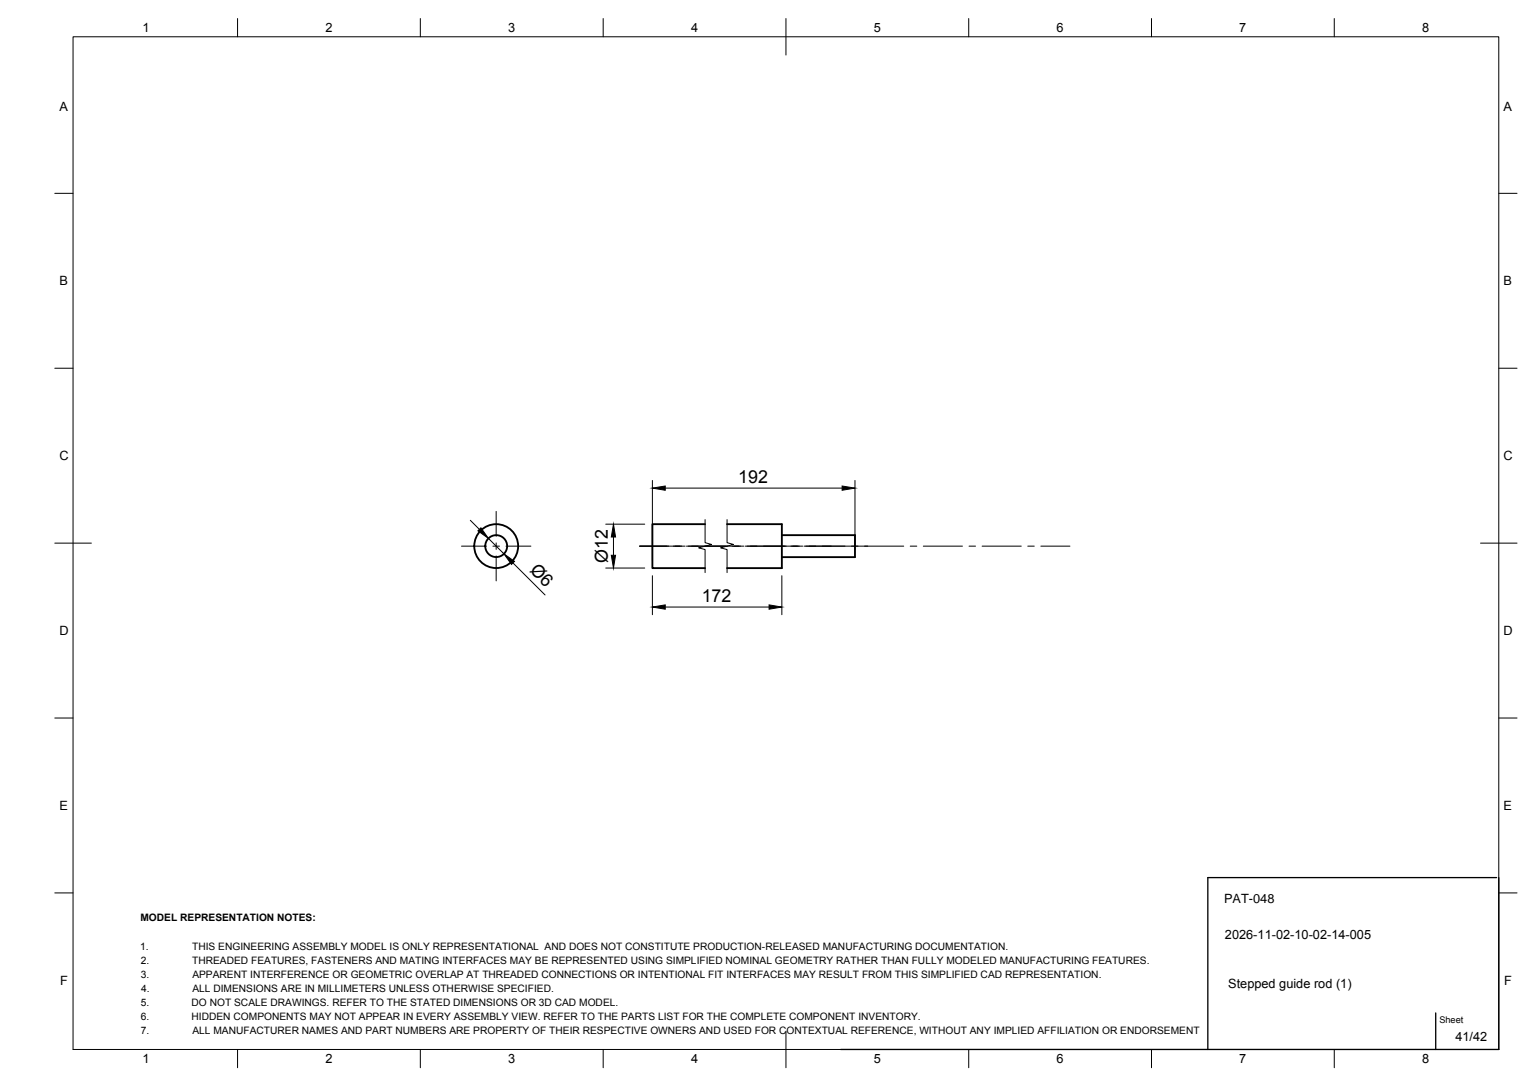
ISO-10303-21;
HEADER;
/* Generated by software containing ST-Developer
 * from STEP Tools, Inc. (www.steptools.com) 
 */

FILE_DESCRIPTION(
/* description */ ('Guided pneumatic stop gate'),
/* implementation_level */ '2;1');

FILE_NAME(
/* name */ 'Stepped guide rod (1).step',
/* time_stamp */ '2026-10-27T21:43:45-07:00',
/* author */ (''),
/* organization */ (''),
/* preprocessor_version */ 'ST-DEVELOPER v20.2',
/* originating_system */ 'Autodesk Translation Framework v15.17.0.0',
/* authorisation */ '');

FILE_SCHEMA (('AUTOMOTIVE_DESIGN { 1 0 10303 214 3 1 1 }'));
ENDSEC;

DATA;
#10=MECHANICAL_DESIGN_GEOMETRIC_PRESENTATION_REPRESENTATION('',(#573),#14392);
#489=SHAPE_REPRESENTATION_RELATIONSHIP('SRR','None',#14626,#531);
#531=ADVANCED_BREP_SHAPE_REPRESENTATION('',(#611),#14388);
#573=STYLED_ITEM('',(#14891),#611);
#611=MANIFOLD_SOLID_BREP('Body1',#7917);
#813=FACE_BOUND('',#2237,.T.);
#1094=PLANE('',#9309);
#1095=PLANE('',#9313);
#1096=PLANE('',#9314);
#1559=FACE_OUTER_BOUND('',#2232,.T.);
#1560=FACE_OUTER_BOUND('',#2233,.T.);
#1561=FACE_OUTER_BOUND('',#2234,.T.);
#1562=FACE_OUTER_BOUND('',#2235,.T.);
#1563=FACE_OUTER_BOUND('',#2236,.T.);
#2232=EDGE_LOOP('',(#7096,#7097,#7098,#7099));
#2233=EDGE_LOOP('',(#7100));
#2234=EDGE_LOOP('',(#7101,#7102,#7103,#7104));
#2235=EDGE_LOOP('',(#7105));
#2236=EDGE_LOOP('',(#7106));
#2237=EDGE_LOOP('',(#7107));
#2783=LINE('',#14104,#3328);
#2784=LINE('',#14111,#3329);
#3328=VECTOR('',#11734,0.3);
#3329=VECTOR('',#11743,0.6);
#3719=CIRCLE('',#9307,0.3);
#3720=CIRCLE('',#9308,0.3);
#3721=CIRCLE('',#9311,0.6);
#3722=CIRCLE('',#9312,0.6);
#4310=VERTEX_POINT('',#14101);
#4311=VERTEX_POINT('',#14103);
#4312=VERTEX_POINT('',#14108);
#4313=VERTEX_POINT('',#14110);
#5246=EDGE_CURVE('',#4310,#4310,#3719,.T.);
#5247=EDGE_CURVE('',#4310,#4311,#2783,.T.);
#5248=EDGE_CURVE('',#4311,#4311,#3720,.T.);
#5249=EDGE_CURVE('',#4312,#4312,#3721,.T.);
#5250=EDGE_CURVE('',#4312,#4313,#2784,.T.);
#5251=EDGE_CURVE('',#4313,#4313,#3722,.T.);
#7096=ORIENTED_EDGE('',*,*,#5246,.F.);
#7097=ORIENTED_EDGE('',*,*,#5247,.T.);
#7098=ORIENTED_EDGE('',*,*,#5248,.T.);
#7099=ORIENTED_EDGE('',*,*,#5247,.F.);
#7100=ORIENTED_EDGE('',*,*,#5248,.F.);
#7101=ORIENTED_EDGE('',*,*,#5249,.F.);
#7102=ORIENTED_EDGE('',*,*,#5250,.T.);
#7103=ORIENTED_EDGE('',*,*,#5251,.T.);
#7104=ORIENTED_EDGE('',*,*,#5250,.F.);
#7105=ORIENTED_EDGE('',*,*,#5249,.T.);
#7106=ORIENTED_EDGE('',*,*,#5251,.F.);
#7107=ORIENTED_EDGE('',*,*,#5246,.T.);
#7392=CYLINDRICAL_SURFACE('',#9306,0.3);
#7393=CYLINDRICAL_SURFACE('',#9310,0.6);
#7841=ADVANCED_FACE('',(#1559),#7392,.T.);
#7842=ADVANCED_FACE('',(#1560),#1094,.F.);
#7843=ADVANCED_FACE('',(#1561),#7393,.T.);
#7844=ADVANCED_FACE('',(#1562),#1095,.T.);
#7845=ADVANCED_FACE('',(#1563,#813),#1096,.F.);
#7917=CLOSED_SHELL('',(#7841,#7842,#7843,#7844,#7845));
#9305=AXIS2_PLACEMENT_3D('',#14099,#11728,#11729);
#9306=AXIS2_PLACEMENT_3D('',#14100,#11730,#11731);
#9307=AXIS2_PLACEMENT_3D('',#14102,#11732,#11733);
#9308=AXIS2_PLACEMENT_3D('',#14105,#11735,#11736);
#9309=AXIS2_PLACEMENT_3D('',#14106,#11737,#11738);
#9310=AXIS2_PLACEMENT_3D('',#14107,#11739,#11740);
#9311=AXIS2_PLACEMENT_3D('',#14109,#11741,#11742);
#9312=AXIS2_PLACEMENT_3D('',#14112,#11744,#11745);
#9313=AXIS2_PLACEMENT_3D('',#14113,#11746,#11747);
#9314=AXIS2_PLACEMENT_3D('',#14114,#11748,#11749);
#11728=DIRECTION('axis',(0.,0.,1.));
#11729=DIRECTION('refdir',(1.,0.,0.));
#11730=DIRECTION('center_axis',(0.,1.,0.));
#11731=DIRECTION('ref_axis',(1.,0.,0.));
#11732=DIRECTION('center_axis',(0.,1.,0.));
#11733=DIRECTION('ref_axis',(1.,0.,0.));
#11734=DIRECTION('',(0.,-1.,0.));
#11735=DIRECTION('center_axis',(0.,1.,0.));
#11736=DIRECTION('ref_axis',(1.,0.,0.));
#11737=DIRECTION('center_axis',(0.,1.,0.));
#11738=DIRECTION('ref_axis',(1.,0.,0.));
#11739=DIRECTION('center_axis',(0.,1.,0.));
#11740=DIRECTION('ref_axis',(1.,0.,0.));
#11741=DIRECTION('center_axis',(0.,1.,0.));
#11742=DIRECTION('ref_axis',(1.,0.,0.));
#11743=DIRECTION('',(0.,-1.,0.));
#11744=DIRECTION('center_axis',(0.,1.,0.));
#11745=DIRECTION('ref_axis',(1.,0.,0.));
#11746=DIRECTION('center_axis',(0.,1.,0.));
#11747=DIRECTION('ref_axis',(1.,0.,0.));
#11748=DIRECTION('center_axis',(0.,1.,0.));
#11749=DIRECTION('ref_axis',(1.,0.,0.));
#14099=CARTESIAN_POINT('',(0.,0.,0.));
#14100=CARTESIAN_POINT('Origin',(5.,-9.4,4.5));
#14101=CARTESIAN_POINT('',(4.7,-7.4,4.5));
#14102=CARTESIAN_POINT('Origin',(5.,-7.4,4.5));
#14103=CARTESIAN_POINT('',(4.7,-9.4,4.5));
#14104=CARTESIAN_POINT('',(4.7,-9.4,4.5));
#14105=CARTESIAN_POINT('Origin',(5.,-9.4,4.5));
#14106=CARTESIAN_POINT('Origin',(5.,-9.4,4.5));
#14107=CARTESIAN_POINT('Origin',(5.,-7.4,4.5));
#14108=CARTESIAN_POINT('',(4.4,9.8,4.5));
#14109=CARTESIAN_POINT('Origin',(5.,9.8,4.5));
#14110=CARTESIAN_POINT('',(4.4,-7.4,4.5));
#14111=CARTESIAN_POINT('',(4.4,-7.4,4.5));
#14112=CARTESIAN_POINT('Origin',(5.,-7.4,4.5));
#14113=CARTESIAN_POINT('Origin',(5.,9.8,4.5));
#14114=CARTESIAN_POINT('Origin',(5.,-7.4,4.5));
#14340=UNCERTAINTY_MEASURE_WITH_UNIT(LENGTH_MEASURE(0.001),#14393,
'DISTANCE_ACCURACY_VALUE',
'Maximum model space distance between geometric entities at asserted c
onnectivities');
#14344=UNCERTAINTY_MEASURE_WITH_UNIT(LENGTH_MEASURE(0.001),#14393,
'DISTANCE_ACCURACY_VALUE',
'Maximum model space distance between geometric entities at asserted c
onnectivities');
#14388=(
GEOMETRIC_REPRESENTATION_CONTEXT(3)
GLOBAL_UNCERTAINTY_ASSIGNED_CONTEXT((#14340))
GLOBAL_UNIT_ASSIGNED_CONTEXT((#14393,#14395,#14396))
REPRESENTATION_CONTEXT('','3D')
);
#14392=(
GEOMETRIC_REPRESENTATION_CONTEXT(3)
GLOBAL_UNCERTAINTY_ASSIGNED_CONTEXT((#14344))
GLOBAL_UNIT_ASSIGNED_CONTEXT((#14393,#14395,#14396))
REPRESENTATION_CONTEXT('','3D')
);
#14393=(
LENGTH_UNIT()
NAMED_UNIT(*)
SI_UNIT(.CENTI.,.METRE.)
);
#14395=(
NAMED_UNIT(*)
PLANE_ANGLE_UNIT()
SI_UNIT($,.RADIAN.)
);
#14396=(
NAMED_UNIT(*)
SI_UNIT($,.STERADIAN.)
SOLID_ANGLE_UNIT()
);
#14440=SHAPE_DEFINITION_REPRESENTATION(#14559,#14626);
#14559=PRODUCT_DEFINITION_SHAPE('',$,#14674);
#14626=SHAPE_REPRESENTATION('',(#9305),#14388);
#14630=PRODUCT_DEFINITION_CONTEXT('part definition',#14773,'design');
#14674=PRODUCT_DEFINITION('Stepped guide rod (1)','Stepped guide rod (1)',
#14721,#14630);
#14721=PRODUCT_DEFINITION_FORMATION('',$,#14818);
#14773=APPLICATION_CONTEXT(
'Core Data for Automotive Mechanical Design Process');
#14774=PRODUCT_CONTEXT('part definition',#14773,'mechanical');
#14818=PRODUCT('Stepped guide rod (1)','Stepped guide rod (1)',
'Stepped guide rod (1)',(#14774));
#14885=COLOUR_RGB('Grey',0.48,0.52,0.57);
#14886=FILL_AREA_STYLE_COLOUR('',#14885);
#14887=FILL_AREA_STYLE('',(#14886));
#14888=SURFACE_STYLE_FILL_AREA(#14887);
#14889=SURFACE_SIDE_STYLE('',(#14888));
#14890=SURFACE_STYLE_USAGE(.BOTH.,#14889);
#14891=PRESENTATION_STYLE_ASSIGNMENT((#14890));
ENDSEC;
END-ISO-10303-21;
